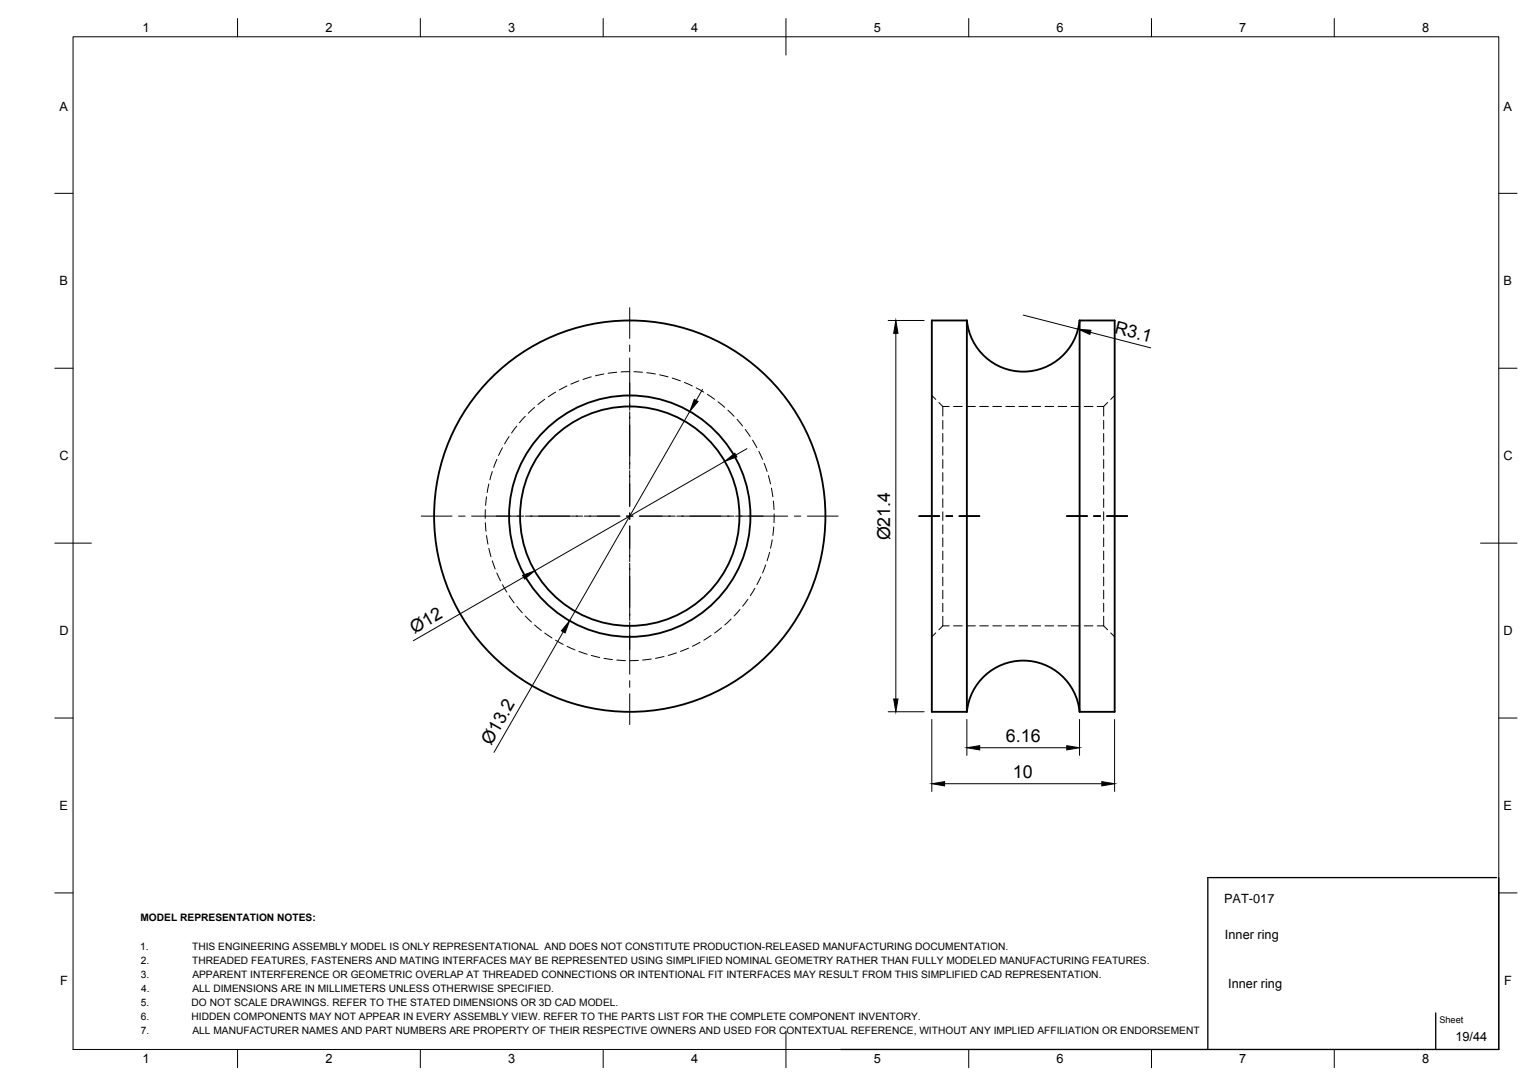
ISO-10303-21;
HEADER;
/* Generated by software containing ST-Developer
 * from STEP Tools, Inc. (www.steptools.com) 
 */

FILE_DESCRIPTION(
/* description */ ('Cam-and-follower valve demonstrator'),
/* implementation_level */ '2;1');

FILE_NAME(
/* name */ 'Inner ring.step',
/* time_stamp */ '2026-10-28T03:25:17-07:00',
/* author */ (''),
/* organization */ (''),
/* preprocessor_version */ 'ST-DEVELOPER v20.2',
/* originating_system */ 'Autodesk Translation Framework v15.17.0.0',
/* authorisation */ '');

FILE_SCHEMA (('AUTOMOTIVE_DESIGN { 1 0 10303 214 3 1 1 }'));
ENDSEC;

DATA;
#10=MECHANICAL_DESIGN_GEOMETRIC_PRESENTATION_REPRESENTATION('',(#424),#12896);
#307=CONICAL_SURFACE('',#6927,0.63,0.785398163397448);
#308=CONICAL_SURFACE('',#6934,0.63,0.785398163397448);
#322=TOROIDAL_SURFACE('',#6916,1.1,0.309556);
#352=SHAPE_REPRESENTATION_RELATIONSHIP('SRR','None',#13069,#388);
#388=ADVANCED_BREP_SHAPE_REPRESENTATION('',(#467),#12869);
#424=STYLED_ITEM('',(#13330),#467);
#467=MANIFOLD_SOLID_BREP('Body1',#6191);
#604=FACE_BOUND('',#1724,.T.);
#605=FACE_BOUND('',#1727,.T.);
#791=CIRCLE('',#6917,1.070235);
#792=CIRCLE('',#6918,1.070235);
#793=CIRCLE('',#6919,0.309556);
#794=CIRCLE('',#6920,1.070235);
#795=CIRCLE('',#6921,1.070235);
#796=CIRCLE('',#6923,1.070235);
#797=CIRCLE('',#6925,0.6);
#798=CIRCLE('',#6926,0.6);
#799=CIRCLE('',#6928,0.66);
#800=CIRCLE('',#6931,1.070235);
#801=CIRCLE('',#6933,0.66);
#1038=CYLINDRICAL_SURFACE('',#6922,1.070235);
#1039=CYLINDRICAL_SURFACE('',#6924,0.6);
#1040=CYLINDRICAL_SURFACE('',#6930,1.070235);
#1242=FACE_OUTER_BOUND('',#1719,.T.);
#1243=FACE_OUTER_BOUND('',#1720,.T.);
#1244=FACE_OUTER_BOUND('',#1721,.T.);
#1245=FACE_OUTER_BOUND('',#1722,.T.);
#1246=FACE_OUTER_BOUND('',#1723,.T.);
#1247=FACE_OUTER_BOUND('',#1725,.T.);
#1248=FACE_OUTER_BOUND('',#1726,.T.);
#1249=FACE_OUTER_BOUND('',#1728,.T.);
#1719=EDGE_LOOP('',(#4755,#4756,#4757,#4758,#4759,#4760));
#1720=EDGE_LOOP('',(#4761,#4762,#4763,#4764,#4765));
#1721=EDGE_LOOP('',(#4766,#4767,#4768,#4769));
#1722=EDGE_LOOP('',(#4770,#4771,#4772,#4773));
#1723=EDGE_LOOP('',(#4774));
#1724=EDGE_LOOP('',(#4775));
#1725=EDGE_LOOP('',(#4776,#4777,#4778,#4779,#4780));
#1726=EDGE_LOOP('',(#4781));
#1727=EDGE_LOOP('',(#4782));
#1728=EDGE_LOOP('',(#4783,#4784,#4785,#4786));
#2192=LINE('',#11507,#2614);
#2193=LINE('',#11513,#2615);
#2194=LINE('',#11517,#2616);
#2195=LINE('',#11523,#2617);
#2196=LINE('',#11528,#2618);
#2614=VECTOR('',#8213,1.070235);
#2615=VECTOR('',#8220,0.6);
#2616=VECTOR('',#8225,0.63);
#2617=VECTOR('',#8234,1.070235);
#2618=VECTOR('',#8241,0.63);
#3059=VERTEX_POINT('',#11496);
#3060=VERTEX_POINT('',#11497);
#3061=VERTEX_POINT('',#11500);
#3062=VERTEX_POINT('',#11502);
#3063=VERTEX_POINT('',#11506);
#3064=VERTEX_POINT('',#11510);
#3065=VERTEX_POINT('',#11512);
#3066=VERTEX_POINT('',#11516);
#3067=VERTEX_POINT('',#11521);
#3068=VERTEX_POINT('',#11525);
#3674=EDGE_CURVE('',#3059,#3060,#791,.T.);
#3675=EDGE_CURVE('',#3060,#3059,#792,.T.);
#3676=EDGE_CURVE('',#3060,#3061,#793,.T.);
#3677=EDGE_CURVE('',#3062,#3061,#794,.T.);
#3678=EDGE_CURVE('',#3061,#3062,#795,.T.);
#3679=EDGE_CURVE('',#3062,#3063,#2192,.T.);
#3680=EDGE_CURVE('',#3063,#3063,#796,.T.);
#3681=EDGE_CURVE('',#3064,#3064,#797,.T.);
#3682=EDGE_CURVE('',#3064,#3065,#2193,.T.);
#3683=EDGE_CURVE('',#3065,#3065,#798,.T.);
#3684=EDGE_CURVE('',#3065,#3066,#2194,.T.);
#3685=EDGE_CURVE('',#3066,#3066,#799,.T.);
#3686=EDGE_CURVE('',#3067,#3067,#800,.T.);
#3687=EDGE_CURVE('',#3067,#3059,#2195,.T.);
#3688=EDGE_CURVE('',#3068,#3068,#801,.T.);
#3689=EDGE_CURVE('',#3068,#3064,#2196,.T.);
#4755=ORIENTED_EDGE('',*,*,#3674,.F.);
#4756=ORIENTED_EDGE('',*,*,#3675,.F.);
#4757=ORIENTED_EDGE('',*,*,#3676,.T.);
#4758=ORIENTED_EDGE('',*,*,#3677,.F.);
#4759=ORIENTED_EDGE('',*,*,#3678,.F.);
#4760=ORIENTED_EDGE('',*,*,#3676,.F.);
#4761=ORIENTED_EDGE('',*,*,#3677,.T.);
#4762=ORIENTED_EDGE('',*,*,#3678,.T.);
#4763=ORIENTED_EDGE('',*,*,#3679,.T.);
#4764=ORIENTED_EDGE('',*,*,#3680,.T.);
#4765=ORIENTED_EDGE('',*,*,#3679,.F.);
#4766=ORIENTED_EDGE('',*,*,#3681,.T.);
#4767=ORIENTED_EDGE('',*,*,#3682,.T.);
#4768=ORIENTED_EDGE('',*,*,#3683,.F.);
#4769=ORIENTED_EDGE('',*,*,#3682,.F.);
#4770=ORIENTED_EDGE('',*,*,#3683,.T.);
#4771=ORIENTED_EDGE('',*,*,#3684,.T.);
#4772=ORIENTED_EDGE('',*,*,#3685,.F.);
#4773=ORIENTED_EDGE('',*,*,#3684,.F.);
#4774=ORIENTED_EDGE('',*,*,#3680,.F.);
#4775=ORIENTED_EDGE('',*,*,#3685,.T.);
#4776=ORIENTED_EDGE('',*,*,#3686,.F.);
#4777=ORIENTED_EDGE('',*,*,#3687,.T.);
#4778=ORIENTED_EDGE('',*,*,#3674,.T.);
#4779=ORIENTED_EDGE('',*,*,#3675,.T.);
#4780=ORIENTED_EDGE('',*,*,#3687,.F.);
#4781=ORIENTED_EDGE('',*,*,#3686,.T.);
#4782=ORIENTED_EDGE('',*,*,#3688,.F.);
#4783=ORIENTED_EDGE('',*,*,#3688,.T.);
#4784=ORIENTED_EDGE('',*,*,#3689,.T.);
#4785=ORIENTED_EDGE('',*,*,#3681,.F.);
#4786=ORIENTED_EDGE('',*,*,#3689,.F.);
#5678=PLANE('',#6929);
#5679=PLANE('',#6932);
#5958=ADVANCED_FACE('',(#1242),#322,.F.);
#5959=ADVANCED_FACE('',(#1243),#1038,.T.);
#5960=ADVANCED_FACE('',(#1244),#1039,.F.);
#5961=ADVANCED_FACE('',(#1245),#307,.F.);
#5962=ADVANCED_FACE('',(#1246,#604),#5678,.T.);
#5963=ADVANCED_FACE('',(#1247),#1040,.T.);
#5964=ADVANCED_FACE('',(#1248,#605),#5679,.T.);
#5965=ADVANCED_FACE('',(#1249),#308,.F.);
#6191=CLOSED_SHELL('',(#5958,#5959,#5960,#5961,#5962,#5963,#5964,#5965));
#6915=AXIS2_PLACEMENT_3D('',#11494,#8197,#8198);
#6916=AXIS2_PLACEMENT_3D('',#11495,#8199,#8200);
#6917=AXIS2_PLACEMENT_3D('',#11498,#8201,#8202);
#6918=AXIS2_PLACEMENT_3D('',#11499,#8203,#8204);
#6919=AXIS2_PLACEMENT_3D('',#11501,#8205,#8206);
#6920=AXIS2_PLACEMENT_3D('',#11503,#8207,#8208);
#6921=AXIS2_PLACEMENT_3D('',#11504,#8209,#8210);
#6922=AXIS2_PLACEMENT_3D('',#11505,#8211,#8212);
#6923=AXIS2_PLACEMENT_3D('',#11508,#8214,#8215);
#6924=AXIS2_PLACEMENT_3D('',#11509,#8216,#8217);
#6925=AXIS2_PLACEMENT_3D('',#11511,#8218,#8219);
#6926=AXIS2_PLACEMENT_3D('',#11514,#8221,#8222);
#6927=AXIS2_PLACEMENT_3D('',#11515,#8223,#8224);
#6928=AXIS2_PLACEMENT_3D('',#11518,#8226,#8227);
#6929=AXIS2_PLACEMENT_3D('',#11519,#8228,#8229);
#6930=AXIS2_PLACEMENT_3D('',#11520,#8230,#8231);
#6931=AXIS2_PLACEMENT_3D('',#11522,#8232,#8233);
#6932=AXIS2_PLACEMENT_3D('',#11524,#8235,#8236);
#6933=AXIS2_PLACEMENT_3D('',#11526,#8237,#8238);
#6934=AXIS2_PLACEMENT_3D('',#11527,#8239,#8240);
#8197=DIRECTION('axis',(0.,0.,1.));
#8198=DIRECTION('refdir',(1.,0.,0.));
#8199=DIRECTION('center_axis',(0.,-1.,0.));
#8200=DIRECTION('ref_axis',(0.,0.,-1.));
#8201=DIRECTION('center_axis',(0.,-1.,0.));
#8202=DIRECTION('ref_axis',(1.,0.,0.));
#8203=DIRECTION('center_axis',(0.,-1.,0.));
#8204=DIRECTION('ref_axis',(1.,0.,0.));
#8205=DIRECTION('center_axis',(1.,0.,1.22464679914735E-16));
#8206=DIRECTION('ref_axis',(-1.22464679914735E-16,0.,1.));
#8207=DIRECTION('center_axis',(0.,1.,0.));
#8208=DIRECTION('ref_axis',(1.,0.,0.));
#8209=DIRECTION('center_axis',(0.,1.,0.));
#8210=DIRECTION('ref_axis',(1.,0.,0.));
#8211=DIRECTION('center_axis',(0.,-1.,0.));
#8212=DIRECTION('ref_axis',(1.,0.,0.));
#8213=DIRECTION('',(0.,1.,0.));
#8214=DIRECTION('center_axis',(0.,-1.,0.));
#8215=DIRECTION('ref_axis',(1.,0.,0.));
#8216=DIRECTION('center_axis',(0.,-1.,0.));
#8217=DIRECTION('ref_axis',(1.,0.,0.));
#8218=DIRECTION('center_axis',(0.,-1.,0.));
#8219=DIRECTION('ref_axis',(1.,0.,0.));
#8220=DIRECTION('',(0.,1.,0.));
#8221=DIRECTION('center_axis',(0.,-1.,0.));
#8222=DIRECTION('ref_axis',(1.,0.,0.));
#8223=DIRECTION('center_axis',(0.,1.,0.));
#8224=DIRECTION('ref_axis',(1.,0.,0.));
#8225=DIRECTION('',(-0.707106781186548,0.707106781186547,-8.65956056235493E-17));
#8226=DIRECTION('center_axis',(0.,-1.,0.));
#8227=DIRECTION('ref_axis',(1.,0.,0.));
#8228=DIRECTION('center_axis',(0.,1.,0.));
#8229=DIRECTION('ref_axis',(0.,0.,1.));
#8230=DIRECTION('center_axis',(0.,-1.,0.));
#8231=DIRECTION('ref_axis',(1.,0.,0.));
#8232=DIRECTION('center_axis',(0.,-1.,0.));
#8233=DIRECTION('ref_axis',(1.,0.,0.));
#8234=DIRECTION('',(0.,1.,0.));
#8235=DIRECTION('center_axis',(0.,-1.,0.));
#8236=DIRECTION('ref_axis',(0.,0.,-1.));
#8237=DIRECTION('center_axis',(0.,-1.,0.));
#8238=DIRECTION('ref_axis',(1.,0.,0.));
#8239=DIRECTION('center_axis',(0.,-1.,0.));
#8240=DIRECTION('ref_axis',(1.,0.,0.));
#8241=DIRECTION('',(0.707106781186548,0.707106781186547,8.65956056235493E-17));
#11494=CARTESIAN_POINT('',(0.,0.,0.));
#11495=CARTESIAN_POINT('Origin',(0.,0.,0.));
#11496=CARTESIAN_POINT('',(-1.070235,-0.308121667383195,-1.31065986708547E-16));
#11497=CARTESIAN_POINT('',(-1.31065986708547E-16,-0.308121667383195,1.070235));
#11498=CARTESIAN_POINT('Origin',(0.,-0.308121667383195,0.));
#11499=CARTESIAN_POINT('Origin',(0.,-0.308121667383195,0.));
#11500=CARTESIAN_POINT('',(-1.31065986708547E-16,0.308121667383195,1.070235));
#11501=CARTESIAN_POINT('Origin',(-1.34711147906209E-16,0.,1.1));
#11502=CARTESIAN_POINT('',(-1.070235,0.308121667383195,1.31065986708547E-16));
#11503=CARTESIAN_POINT('Origin',(0.,0.308121667383195,0.));
#11504=CARTESIAN_POINT('Origin',(0.,0.308121667383195,0.));
#11505=CARTESIAN_POINT('Origin',(0.,0.,0.));
#11506=CARTESIAN_POINT('',(-1.070235,0.5,-1.31065986708547E-16));
#11507=CARTESIAN_POINT('',(-1.070235,0.,-1.31065986708547E-16));
#11508=CARTESIAN_POINT('Origin',(0.,0.5,0.));
#11509=CARTESIAN_POINT('Origin',(0.,0.,0.));
#11510=CARTESIAN_POINT('',(-0.6,-0.44,-7.34788079488412E-17));
#11511=CARTESIAN_POINT('Origin',(0.,-0.44,0.));
#11512=CARTESIAN_POINT('',(-0.6,0.44,-7.34788079488412E-17));
#11513=CARTESIAN_POINT('',(-0.6,0.,-7.34788079488412E-17));
#11514=CARTESIAN_POINT('Origin',(0.,0.44,0.));
#11515=CARTESIAN_POINT('Origin',(0.,0.47,0.));
#11516=CARTESIAN_POINT('',(-0.66,0.5,-8.08266887437253E-17));
#11517=CARTESIAN_POINT('',(-0.63,0.47,-7.71527483462832E-17));
#11518=CARTESIAN_POINT('Origin',(0.,0.5,0.));
#11519=CARTESIAN_POINT('Origin',(1.070235,0.5,0.));
#11520=CARTESIAN_POINT('Origin',(0.,0.,0.));
#11521=CARTESIAN_POINT('',(-1.070235,-0.5,-1.31065986708547E-16));
#11522=CARTESIAN_POINT('Origin',(0.,-0.5,0.));
#11523=CARTESIAN_POINT('',(-1.070235,0.,-1.31065986708547E-16));
#11524=CARTESIAN_POINT('Origin',(0.66,-0.5,0.));
#11525=CARTESIAN_POINT('',(-0.66,-0.5,-8.08266887437253E-17));
#11526=CARTESIAN_POINT('Origin',(0.,-0.5,0.));
#11527=CARTESIAN_POINT('Origin',(0.,-0.47,0.));
#11528=CARTESIAN_POINT('',(-0.63,-0.47,-7.71527483462832E-17));
#12826=UNCERTAINTY_MEASURE_WITH_UNIT(LENGTH_MEASURE(0.001),#12897,
'DISTANCE_ACCURACY_VALUE',
'Maximum model space distance between geometric entities at asserted c
onnectivities');
#12853=UNCERTAINTY_MEASURE_WITH_UNIT(LENGTH_MEASURE(0.001),#12897,
'DISTANCE_ACCURACY_VALUE',
'Maximum model space distance between geometric entities at asserted c
onnectivities');
#12869=(
GEOMETRIC_REPRESENTATION_CONTEXT(3)
GLOBAL_UNCERTAINTY_ASSIGNED_CONTEXT((#12826))
GLOBAL_UNIT_ASSIGNED_CONTEXT((#12897,#12899,#12900))
REPRESENTATION_CONTEXT('','3D')
);
#12896=(
GEOMETRIC_REPRESENTATION_CONTEXT(3)
GLOBAL_UNCERTAINTY_ASSIGNED_CONTEXT((#12853))
GLOBAL_UNIT_ASSIGNED_CONTEXT((#12897,#12899,#12900))
REPRESENTATION_CONTEXT('','3D')
);
#12897=(
LENGTH_UNIT()
NAMED_UNIT(*)
SI_UNIT(.CENTI.,.METRE.)
);
#12899=(
NAMED_UNIT(*)
PLANE_ANGLE_UNIT()
SI_UNIT($,.RADIAN.)
);
#12900=(
NAMED_UNIT(*)
SI_UNIT($,.STERADIAN.)
SOLID_ANGLE_UNIT()
);
#12916=SHAPE_DEFINITION_REPRESENTATION(#12958,#13069);
#12958=PRODUCT_DEFINITION_SHAPE('',$,#13112);
#13069=SHAPE_REPRESENTATION('',(#6915),#12869);
#13096=PRODUCT_DEFINITION_CONTEXT('part definition',#13224,'design');
#13112=PRODUCT_DEFINITION('Inner ring','Inner ring',#13154,#13096);
#13154=PRODUCT_DEFINITION_FORMATION('',$,#13241);
#13224=APPLICATION_CONTEXT(
'Core Data for Automotive Mechanical Design Process');
#13225=PRODUCT_CONTEXT('part definition',#13224,'mechanical');
#13241=PRODUCT('Inner ring','Inner ring','Inner ring',(#13225));
#13324=COLOUR_RGB('Grey',0.48,0.52,0.57);
#13325=FILL_AREA_STYLE_COLOUR('',#13324);
#13326=FILL_AREA_STYLE('',(#13325));
#13327=SURFACE_STYLE_FILL_AREA(#13326);
#13328=SURFACE_SIDE_STYLE('',(#13327));
#13329=SURFACE_STYLE_USAGE(.BOTH.,#13328);
#13330=PRESENTATION_STYLE_ASSIGNMENT((#13329));
ENDSEC;
END-ISO-10303-21;
